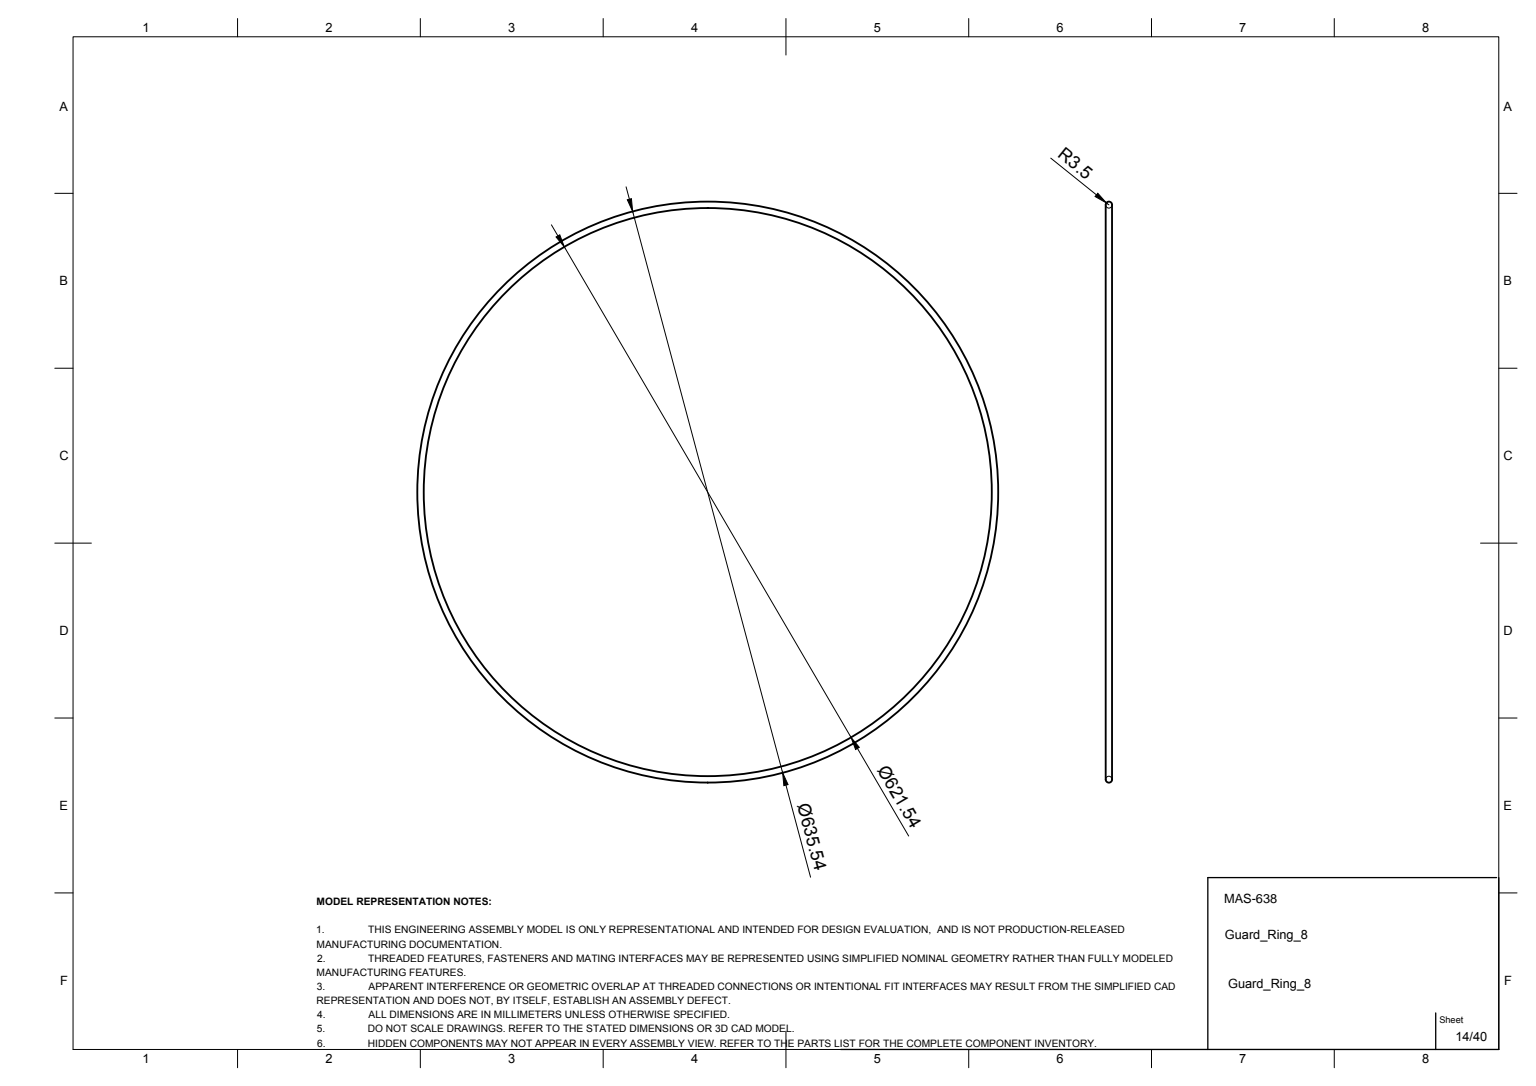
ISO-10303-21;
HEADER;
FILE_DESCRIPTION((''),'2;1');
FILE_NAME('Guard_Ring_8.step','2026-10-09T12:00:21-07:00',(''),(''),'','','');
FILE_SCHEMA (('AUTOMOTIVE_DESIGN { 1 0 10303 214 3 1 1 }'));
ENDSEC;
DATA;
#10=MECHANICAL_DESIGN_GEOMETRIC_PRESENTATION_REPRESENTATION('',(#405,#406),#10334);
#341=SHAPE_REPRESENTATION_RELATIONSHIP('SRR','None',#10457,#373) ;
#373=ADVANCED_BREP_SHAPE_REPRESENTATION('',(#445),#10309) ;
#405=STYLED_ITEM('',(#10631),#3374) ;
#406=STYLED_ITEM('',(#10632),#445) ;
#445=MANIFOLD_SOLID_BREP('Body1',#3567) ;
#866=FACE_OUTER_BOUND('',#1066,.T.) ;
#1066=EDGE_LOOP('',(#2377,#2378,#2379,#2380)) ;
#1290=CIRCLE('',#4003,0.349999999999999) ;
#1291=CIRCLE('',#4004,31.0768144613668) ;
#1520=VERTEX_POINT('',#5688) ;
#1845=EDGE_CURVE('',#1520,#1520,#1290,.T.) ;
#1846=EDGE_CURVE('',#1520,#1520,#1291,.T.) ;
#2377=ORIENTED_EDGE('',*,*,#1845,.F.) ;
#2378=ORIENTED_EDGE('',*,*,#1846,.T.) ;
#2379=ORIENTED_EDGE('',*,*,#1845,.T.) ;
#2380=ORIENTED_EDGE('',*,*,#1846,.F.) ;
#3312=TOROIDAL_SURFACE('',#4002,31.4268144613668,0.349999999999999) ;
#3374=ADVANCED_FACE('',(#866),#3312,.T.) ;
#3567=CLOSED_SHELL('',(#3374)) ;
#4001=AXIS2_PLACEMENT_3D('',#5686,#4563,#4564) ;
#4002=AXIS2_PLACEMENT_3D('',#5687,#4565,#4566) ;
#4003=AXIS2_PLACEMENT_3D('',#5689,#4567,#4568) ;
#4004=AXIS2_PLACEMENT_3D('',#5690,#4569,#4570) ;
#4563=DIRECTION('axis',(0.,0.,1.)) ;
#4564=DIRECTION('refdir',(1.,0.,0.)) ;
#4565=DIRECTION('center_axis',(-6.42891162084177E-17,-1.,-1.01883556321148E-16)) ;
#4566=DIRECTION('ref_axis',(1.,0.,0.)) ;
#4567=DIRECTION('center_axis',(0.,1.01883556321148E-16,-1.)) ;
#4568=DIRECTION('ref_axis',(-1.,0.,0.)) ;
#4569=DIRECTION('center_axis',(6.42891162084177E-17,1.,1.01883556321148E-16)) ;
#4570=DIRECTION('ref_axis',(1.,-6.42891162084177E-17,-6.55000379205715E-33)) ;
#5686=CARTESIAN_POINT('',(0.,0.,0.)) ;
#5687=CARTESIAN_POINT('Origin',(23.47768801576,67.3831179463143,68.2224337400009)) ;
#5688=CARTESIAN_POINT('',(-7.5991264456068,67.3831179463143,68.2224337400009)) ;
#5689=CARTESIAN_POINT('Origin',(-7.9491264456068,67.3831179463143,68.2224337400009)) ;
#5690=CARTESIAN_POINT('Origin',(23.47768801576,67.3831179463143,68.2224337400009)) ;
#10272=UNCERTAINTY_MEASURE_WITH_UNIT(LENGTH_MEASURE(0.001),#10335,
'DISTANCE_ACCURACY_VALUE',
'Maximum model space distance between geometric entities at asserted c
onnectivities') ;
#10297=UNCERTAINTY_MEASURE_WITH_UNIT(LENGTH_MEASURE(0.001),#10335,
'DISTANCE_ACCURACY_VALUE',
'Maximum model space distance between geometric entities at asserted c
onnectivities') ;
#10309=(
GEOMETRIC_REPRESENTATION_CONTEXT(3)
GLOBAL_UNCERTAINTY_ASSIGNED_CONTEXT((#10272))
GLOBAL_UNIT_ASSIGNED_CONTEXT((#10335,#10337,#10338))
REPRESENTATION_CONTEXT('','3D')
) ;
#10334=(
GEOMETRIC_REPRESENTATION_CONTEXT(3)
GLOBAL_UNCERTAINTY_ASSIGNED_CONTEXT((#10297))
GLOBAL_UNIT_ASSIGNED_CONTEXT((#10335,#10337,#10338))
REPRESENTATION_CONTEXT('','3D')
) ;
#10335=(
LENGTH_UNIT()
NAMED_UNIT(*)
SI_UNIT(.CENTI.,.METRE.)
) ;
#10337=(
NAMED_UNIT(*)
PLANE_ANGLE_UNIT()
SI_UNIT($,.RADIAN.)
) ;
#10338=(
NAMED_UNIT(*)
SI_UNIT($,.STERADIAN.)
SOLID_ANGLE_UNIT()
) ;
#10350=SHAPE_DEFINITION_REPRESENTATION(#10386,#10457) ;
#10386=PRODUCT_DEFINITION_SHAPE('',$,#10494) ;
#10457=SHAPE_REPRESENTATION('',(#4001),#10309) ;
#10482=PRODUCT_DEFINITION_CONTEXT('part definition',#10592,'design') ;
#10494=PRODUCT_DEFINITION('Guard_Ring_8','Guard_Ring_8',#10530,#10482) ;
#10530=PRODUCT_DEFINITION_FORMATION('',$,#10605) ;
#10592=APPLICATION_CONTEXT(
'Core Data for Automotive Mechanical Design Process') ;
#10593=PRODUCT_CONTEXT('part definition',#10592,'mechanical') ;
#10605=PRODUCT('Guard_Ring_8','Guard_Ring_8',$,(#10593)) ;
#10631=PRESENTATION_STYLE_ASSIGNMENT((#10635)) ;
#10632=PRESENTATION_STYLE_ASSIGNMENT((#10636)) ;
#10635=SURFACE_STYLE_USAGE(.BOTH.,#10639) ;
#10636=SURFACE_STYLE_USAGE(.BOTH.,#10640) ;
#10639=SURFACE_SIDE_STYLE('',(#10643)) ;
#10640=SURFACE_SIDE_STYLE('',(#10644)) ;
#10643=SURFACE_STYLE_FILL_AREA(#10647) ;
#10644=SURFACE_STYLE_FILL_AREA(#10648) ;
#10647=FILL_AREA_STYLE('Opaque(25,25,25)',(#10651)) ;
#10648=FILL_AREA_STYLE('Opaque(202,209,238)',(#10652)) ;
#10651=FILL_AREA_STYLE_COLOUR('Opaque(25,25,25)',#10655) ;
#10652=FILL_AREA_STYLE_COLOUR('Opaque(202,209,238)',#10656) ;
#10655=COLOUR_RGB('Opaque(25,25,25)', 0.09019608, 0.27058824, 0.51372549) ;
#10656=COLOUR_RGB('Opaque(202,209,238)', 0.40784314, 0.44705882, 0.49803922) ;
ENDSEC;
END-ISO-10303-21;
